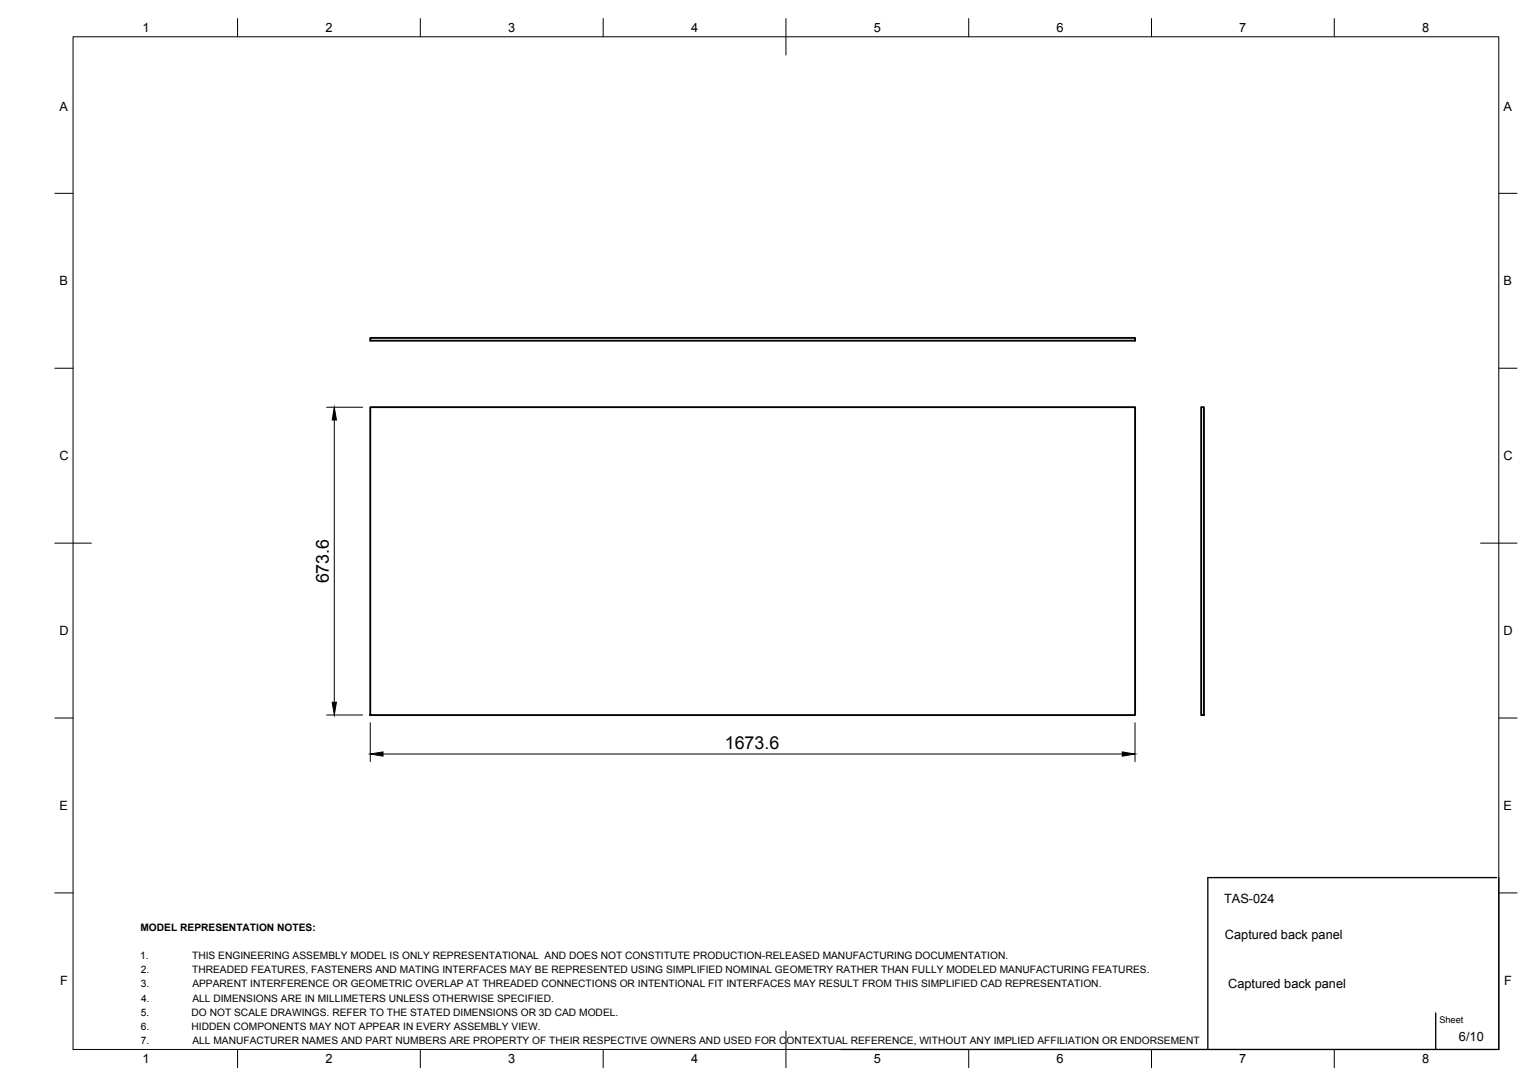
ISO-10303-21;
HEADER;
/* Generated by software containing ST-Developer
 * from STEP Tools, Inc. (www.steptools.com) 
 */

FILE_DESCRIPTION(
/* description */ (''),
/* implementation_level */ '2;1');

FILE_NAME(
/* name */ 'Captured back panel.step',
/* time_stamp */ '2026-11-15T17:53:25-08:00',
/* author */ (''),
/* organization */ (''),
/* preprocessor_version */ 'ST-DEVELOPER v20.2',
/* originating_system */ 'Autodesk Translation Framework v15.17.0.0',
/* authorisation */ '');

FILE_SCHEMA (('AUTOMOTIVE_DESIGN { 1 0 10303 214 3 1 1 }'));
ENDSEC;

DATA;
#10=MECHANICAL_DESIGN_GEOMETRIC_PRESENTATION_REPRESENTATION('',(#134),#2673);
#118=SHAPE_REPRESENTATION_RELATIONSHIP('SRR','None',#2726,#126);
#126=ADVANCED_BREP_SHAPE_REPRESENTATION('',(#142),#2668);
#134=STYLED_ITEM('',(#2775),#142);
#142=MANIFOLD_SOLID_BREP('Body1',#1520);
#212=PLANE('',#1701);
#213=PLANE('',#1702);
#214=PLANE('',#1703);
#215=PLANE('',#1704);
#216=PLANE('',#1705);
#217=PLANE('',#1706);
#295=FACE_OUTER_BOUND('',#394,.T.);
#296=FACE_OUTER_BOUND('',#395,.T.);
#297=FACE_OUTER_BOUND('',#396,.T.);
#298=FACE_OUTER_BOUND('',#397,.T.);
#299=FACE_OUTER_BOUND('',#398,.T.);
#300=FACE_OUTER_BOUND('',#399,.T.);
#394=EDGE_LOOP('',(#1328,#1329,#1330,#1331));
#395=EDGE_LOOP('',(#1332,#1333,#1334,#1335));
#396=EDGE_LOOP('',(#1336,#1337,#1338,#1339));
#397=EDGE_LOOP('',(#1340,#1341,#1342,#1343));
#398=EDGE_LOOP('',(#1344,#1345,#1346,#1347));
#399=EDGE_LOOP('',(#1348,#1349,#1350,#1351));
#542=LINE('',#2530,#690);
#543=LINE('',#2532,#691);
#544=LINE('',#2534,#692);
#545=LINE('',#2535,#693);
#546=LINE('',#2538,#694);
#547=LINE('',#2540,#695);
#548=LINE('',#2541,#696);
#549=LINE('',#2544,#697);
#550=LINE('',#2546,#698);
#551=LINE('',#2547,#699);
#552=LINE('',#2549,#700);
#553=LINE('',#2550,#701);
#690=VECTOR('',#2064,1.);
#691=VECTOR('',#2065,1.);
#692=VECTOR('',#2066,1.);
#693=VECTOR('',#2067,1.);
#694=VECTOR('',#2070,1.);
#695=VECTOR('',#2071,1.);
#696=VECTOR('',#2072,1.);
#697=VECTOR('',#2075,1.);
#698=VECTOR('',#2076,1.);
#699=VECTOR('',#2077,1.);
#700=VECTOR('',#2080,1.);
#701=VECTOR('',#2081,1.);
#844=VERTEX_POINT('',#2528);
#845=VERTEX_POINT('',#2529);
#846=VERTEX_POINT('',#2531);
#847=VERTEX_POINT('',#2533);
#848=VERTEX_POINT('',#2537);
#849=VERTEX_POINT('',#2539);
#850=VERTEX_POINT('',#2543);
#851=VERTEX_POINT('',#2545);
#1010=EDGE_CURVE('',#844,#845,#542,.T.);
#1011=EDGE_CURVE('',#845,#846,#543,.T.);
#1012=EDGE_CURVE('',#847,#846,#544,.T.);
#1013=EDGE_CURVE('',#844,#847,#545,.T.);
#1014=EDGE_CURVE('',#848,#844,#546,.T.);
#1015=EDGE_CURVE('',#849,#847,#547,.T.);
#1016=EDGE_CURVE('',#848,#849,#548,.T.);
#1017=EDGE_CURVE('',#850,#848,#549,.T.);
#1018=EDGE_CURVE('',#851,#849,#550,.T.);
#1019=EDGE_CURVE('',#850,#851,#551,.T.);
#1020=EDGE_CURVE('',#845,#850,#552,.T.);
#1021=EDGE_CURVE('',#846,#851,#553,.T.);
#1328=ORIENTED_EDGE('',*,*,#1010,.T.);
#1329=ORIENTED_EDGE('',*,*,#1011,.T.);
#1330=ORIENTED_EDGE('',*,*,#1012,.F.);
#1331=ORIENTED_EDGE('',*,*,#1013,.F.);
#1332=ORIENTED_EDGE('',*,*,#1014,.T.);
#1333=ORIENTED_EDGE('',*,*,#1013,.T.);
#1334=ORIENTED_EDGE('',*,*,#1015,.F.);
#1335=ORIENTED_EDGE('',*,*,#1016,.F.);
#1336=ORIENTED_EDGE('',*,*,#1017,.T.);
#1337=ORIENTED_EDGE('',*,*,#1016,.T.);
#1338=ORIENTED_EDGE('',*,*,#1018,.F.);
#1339=ORIENTED_EDGE('',*,*,#1019,.F.);
#1340=ORIENTED_EDGE('',*,*,#1020,.T.);
#1341=ORIENTED_EDGE('',*,*,#1019,.T.);
#1342=ORIENTED_EDGE('',*,*,#1021,.F.);
#1343=ORIENTED_EDGE('',*,*,#1011,.F.);
#1344=ORIENTED_EDGE('',*,*,#1021,.T.);
#1345=ORIENTED_EDGE('',*,*,#1018,.T.);
#1346=ORIENTED_EDGE('',*,*,#1015,.T.);
#1347=ORIENTED_EDGE('',*,*,#1012,.T.);
#1348=ORIENTED_EDGE('',*,*,#1020,.F.);
#1349=ORIENTED_EDGE('',*,*,#1010,.F.);
#1350=ORIENTED_EDGE('',*,*,#1014,.F.);
#1351=ORIENTED_EDGE('',*,*,#1017,.F.);
#1490=ADVANCED_FACE('',(#295),#212,.T.);
#1491=ADVANCED_FACE('',(#296),#213,.T.);
#1492=ADVANCED_FACE('',(#297),#214,.T.);
#1493=ADVANCED_FACE('',(#298),#215,.T.);
#1494=ADVANCED_FACE('',(#299),#216,.T.);
#1495=ADVANCED_FACE('',(#300),#217,.F.);
#1520=CLOSED_SHELL('',(#1490,#1491,#1492,#1493,#1494,#1495));
#1700=AXIS2_PLACEMENT_3D('',#2526,#2060,#2061);
#1701=AXIS2_PLACEMENT_3D('',#2527,#2062,#2063);
#1702=AXIS2_PLACEMENT_3D('',#2536,#2068,#2069);
#1703=AXIS2_PLACEMENT_3D('',#2542,#2073,#2074);
#1704=AXIS2_PLACEMENT_3D('',#2548,#2078,#2079);
#1705=AXIS2_PLACEMENT_3D('',#2551,#2082,#2083);
#1706=AXIS2_PLACEMENT_3D('',#2552,#2084,#2085);
#2060=DIRECTION('axis',(0.,0.,1.));
#2061=DIRECTION('refdir',(1.,0.,0.));
#2062=DIRECTION('center_axis',(0.,1.,0.));
#2063=DIRECTION('ref_axis',(-1.,0.,0.));
#2064=DIRECTION('',(-1.,0.,0.));
#2065=DIRECTION('',(0.,0.,1.));
#2066=DIRECTION('',(-1.,0.,0.));
#2067=DIRECTION('',(0.,0.,1.));
#2068=DIRECTION('center_axis',(1.,0.,0.));
#2069=DIRECTION('ref_axis',(0.,1.,0.));
#2070=DIRECTION('',(0.,1.,0.));
#2071=DIRECTION('',(0.,1.,0.));
#2072=DIRECTION('',(0.,0.,1.));
#2073=DIRECTION('center_axis',(0.,-1.,0.));
#2074=DIRECTION('ref_axis',(1.,0.,0.));
#2075=DIRECTION('',(1.,0.,0.));
#2076=DIRECTION('',(1.,0.,0.));
#2077=DIRECTION('',(0.,0.,1.));
#2078=DIRECTION('center_axis',(-1.,0.,0.));
#2079=DIRECTION('ref_axis',(0.,-1.,0.));
#2080=DIRECTION('',(0.,-1.,0.));
#2081=DIRECTION('',(0.,-1.,0.));
#2082=DIRECTION('center_axis',(0.,0.,1.));
#2083=DIRECTION('ref_axis',(1.,0.,0.));
#2084=DIRECTION('center_axis',(0.,0.,1.));
#2085=DIRECTION('ref_axis',(1.,0.,0.));
#2526=CARTESIAN_POINT('',(0.,0.,0.));
#2527=CARTESIAN_POINT('Origin',(67.36,0.6,0.));
#2528=CARTESIAN_POINT('',(67.36,0.6,0.));
#2529=CARTESIAN_POINT('',(0.,0.6,0.));
#2530=CARTESIAN_POINT('',(67.36,0.6,0.));
#2531=CARTESIAN_POINT('',(0.,0.6,167.36));
#2532=CARTESIAN_POINT('',(0.,0.6,0.));
#2533=CARTESIAN_POINT('',(67.36,0.6,167.36));
#2534=CARTESIAN_POINT('',(67.36,0.6,167.36));
#2535=CARTESIAN_POINT('',(67.36,0.6,0.));
#2536=CARTESIAN_POINT('Origin',(67.36,0.,0.));
#2537=CARTESIAN_POINT('',(67.36,0.,0.));
#2538=CARTESIAN_POINT('',(67.36,0.,0.));
#2539=CARTESIAN_POINT('',(67.36,0.,167.36));
#2540=CARTESIAN_POINT('',(67.36,0.,167.36));
#2541=CARTESIAN_POINT('',(67.36,0.,0.));
#2542=CARTESIAN_POINT('Origin',(0.,0.,0.));
#2543=CARTESIAN_POINT('',(0.,0.,0.));
#2544=CARTESIAN_POINT('',(0.,0.,0.));
#2545=CARTESIAN_POINT('',(0.,0.,167.36));
#2546=CARTESIAN_POINT('',(0.,0.,167.36));
#2547=CARTESIAN_POINT('',(0.,0.,0.));
#2548=CARTESIAN_POINT('Origin',(0.,0.6,0.));
#2549=CARTESIAN_POINT('',(0.,0.6,0.));
#2550=CARTESIAN_POINT('',(0.,0.6,167.36));
#2551=CARTESIAN_POINT('Origin',(33.68,0.3,167.36));
#2552=CARTESIAN_POINT('Origin',(33.68,0.3,0.));
#2658=UNCERTAINTY_MEASURE_WITH_UNIT(LENGTH_MEASURE(0.001),#2674,
'DISTANCE_ACCURACY_VALUE',
'Maximum model space distance between geometric entities at asserted c
onnectivities');
#2663=UNCERTAINTY_MEASURE_WITH_UNIT(LENGTH_MEASURE(0.001),#2674,
'DISTANCE_ACCURACY_VALUE',
'Maximum model space distance between geometric entities at asserted c
onnectivities');
#2668=(
GEOMETRIC_REPRESENTATION_CONTEXT(3)
GLOBAL_UNCERTAINTY_ASSIGNED_CONTEXT((#2658))
GLOBAL_UNIT_ASSIGNED_CONTEXT((#2674,#2676,#2677))
REPRESENTATION_CONTEXT('','3D')
);
#2673=(
GEOMETRIC_REPRESENTATION_CONTEXT(3)
GLOBAL_UNCERTAINTY_ASSIGNED_CONTEXT((#2663))
GLOBAL_UNIT_ASSIGNED_CONTEXT((#2674,#2676,#2677))
REPRESENTATION_CONTEXT('','3D')
);
#2674=(
LENGTH_UNIT()
NAMED_UNIT(*)
SI_UNIT(.CENTI.,.METRE.)
);
#2676=(
NAMED_UNIT(*)
PLANE_ANGLE_UNIT()
SI_UNIT($,.RADIAN.)
);
#2677=(
NAMED_UNIT(*)
SI_UNIT($,.STERADIAN.)
SOLID_ANGLE_UNIT()
);
#2682=SHAPE_DEFINITION_REPRESENTATION(#2691,#2726);
#2691=PRODUCT_DEFINITION_SHAPE('',$,#2736);
#2726=SHAPE_REPRESENTATION('',(#1700),#2668);
#2731=PRODUCT_DEFINITION_CONTEXT('part definition',#2760,'design');
#2736=PRODUCT_DEFINITION('Captured back panel','Captured back panel',#2745,
#2731);
#2745=PRODUCT_DEFINITION_FORMATION('',$,#2766);
#2760=APPLICATION_CONTEXT(
'Core Data for Automotive Mechanical Design Process');
#2761=PRODUCT_CONTEXT('part definition',#2760,'mechanical');
#2766=PRODUCT('Captured back panel','Captured back panel',$,(#2761));
#2775=PRESENTATION_STYLE_ASSIGNMENT((#2784));
#2784=SURFACE_STYLE_USAGE(.BOTH.,#2793);
#2793=SURFACE_SIDE_STYLE('',(#2802));
#2802=SURFACE_STYLE_FILL_AREA(#2811);
#2811=FILL_AREA_STYLE('Captured back panel finish',(#2820));
#2820=FILL_AREA_STYLE_COLOUR('Captured back panel finish',#2829);
#2829=COLOUR_RGB('Captured back panel finish',0.607843137254902,0.647058823529412,
0.701960784313725);
ENDSEC;
END-ISO-10303-21;
